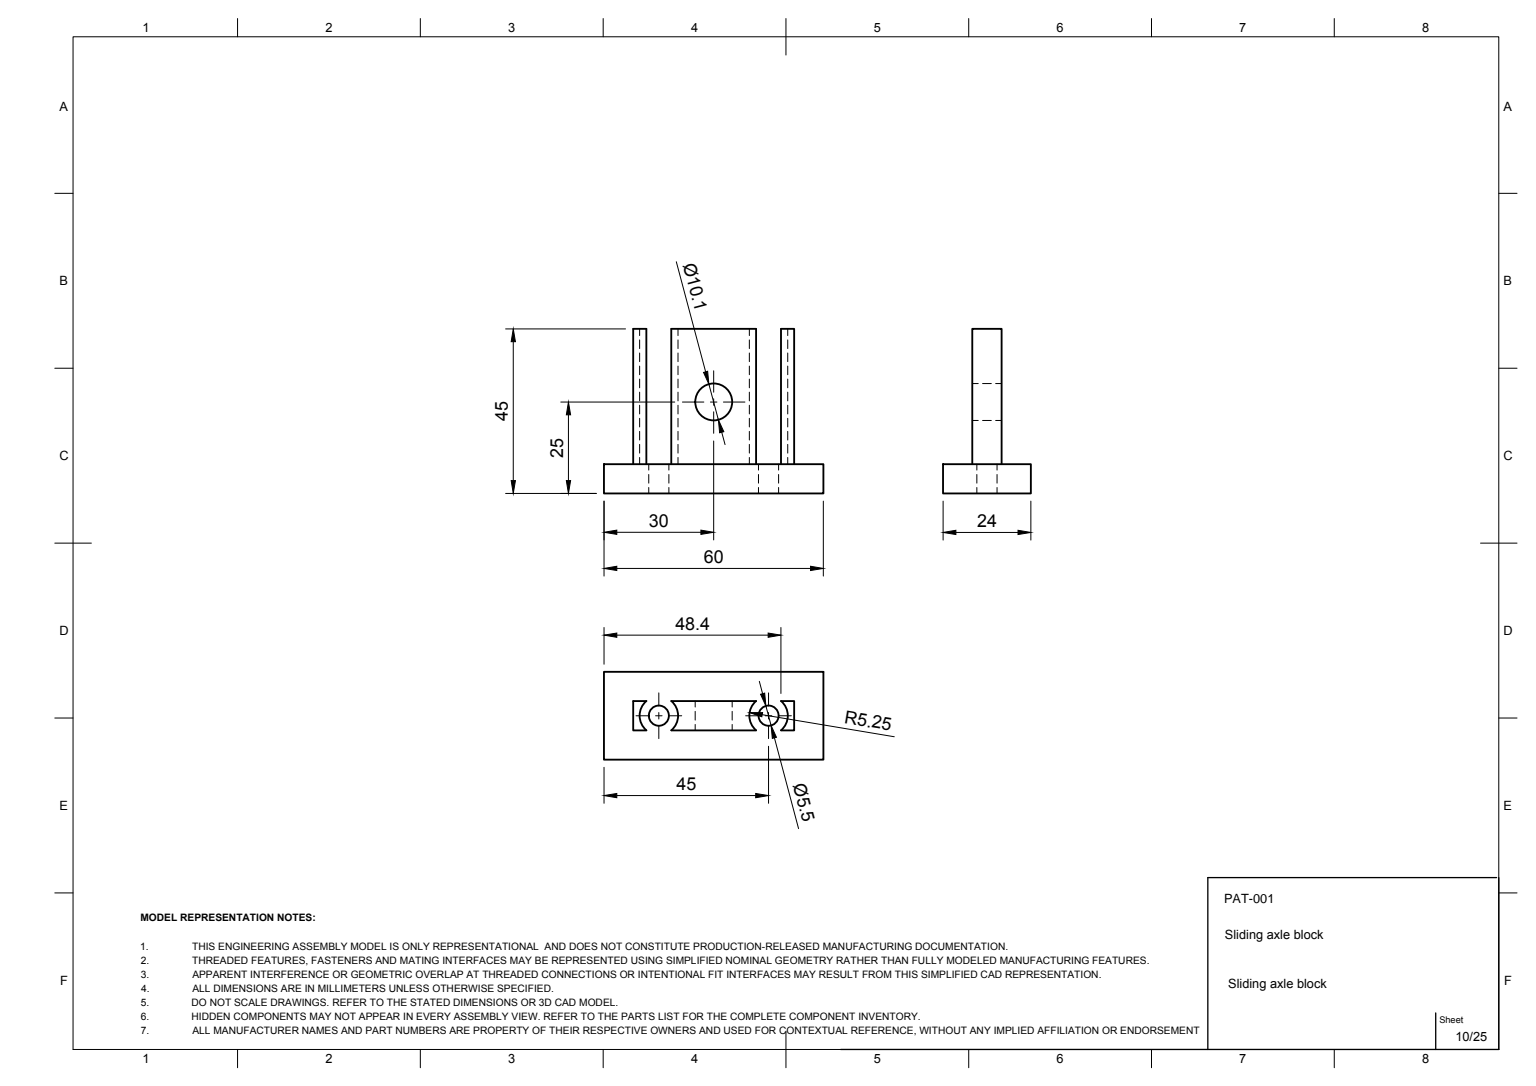
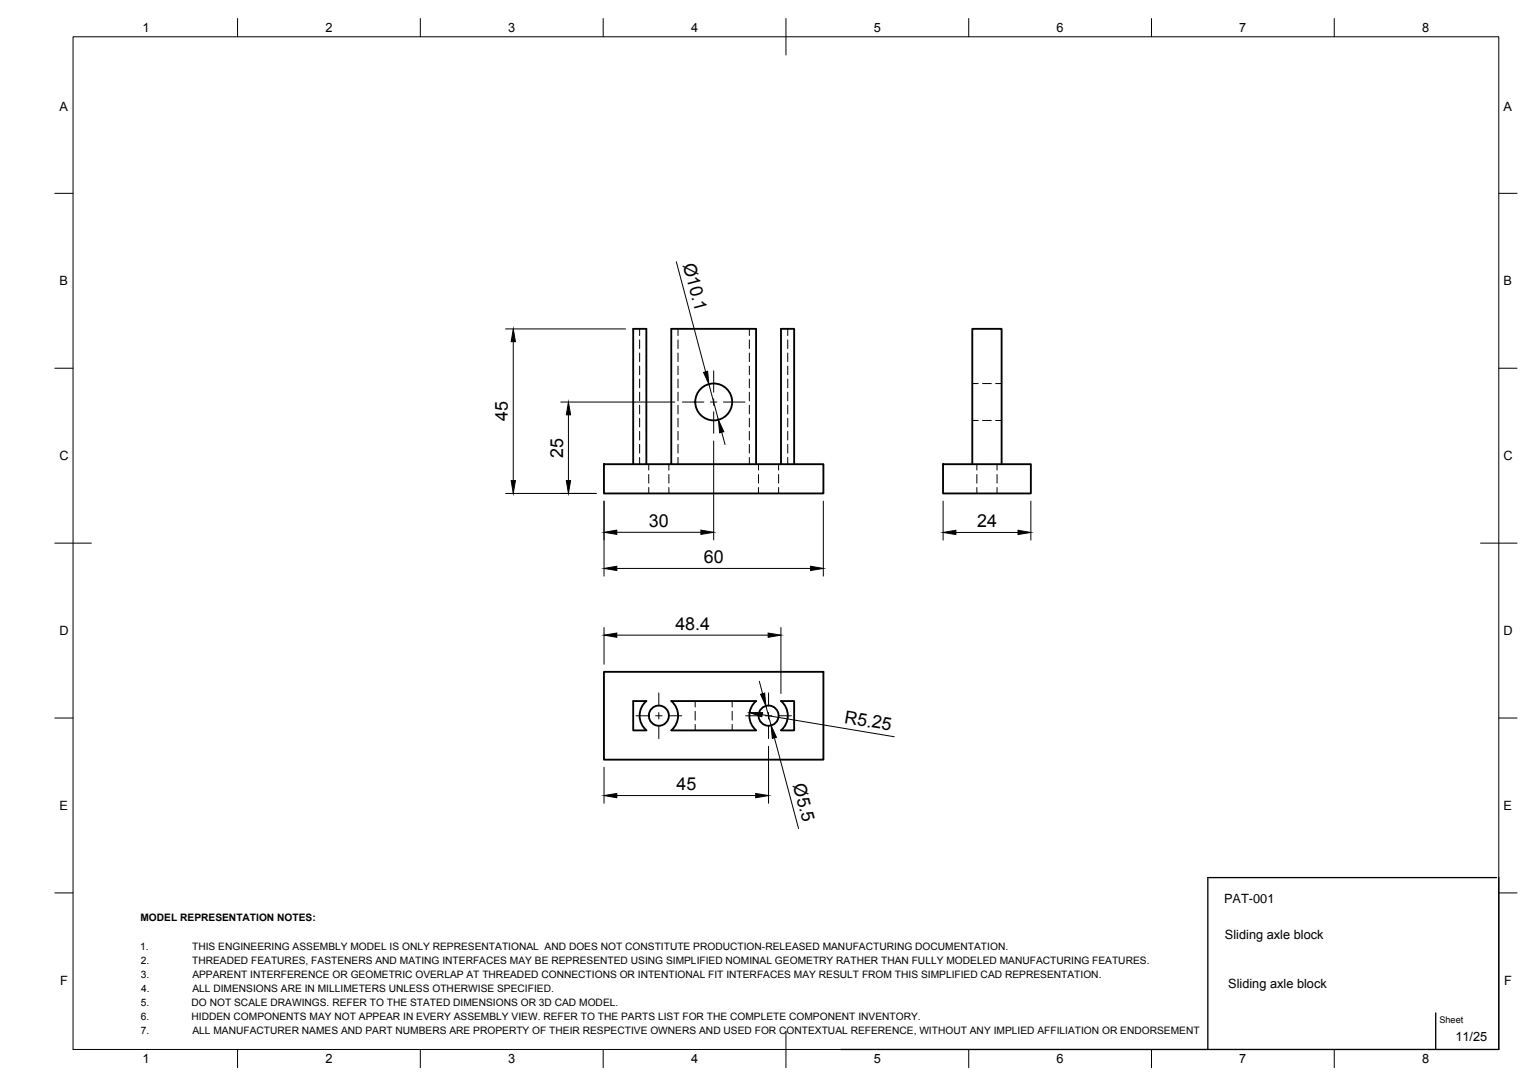
ISO-10303-21;
HEADER;
/* Generated by software containing ST-Developer
 * from STEP Tools, Inc. (www.steptools.com) 
 */

FILE_DESCRIPTION(
/* description */ ('PAT-001'),
/* implementation_level */ '2;1');

FILE_NAME(
/* name */ 'Sliding axle block.step',
/* time_stamp */ '2026-10-29T17:07:15-07:00',
/* author */ (''),
/* organization */ (''),
/* preprocessor_version */ 'ST-DEVELOPER v20.2',
/* originating_system */ 'Autodesk Translation Framework v15.17.0.0',
/* authorisation */ '');

FILE_SCHEMA (('AUTOMOTIVE_DESIGN { 1 0 10303 214 3 1 1 }'));
ENDSEC;

DATA;
#10=MECHANICAL_DESIGN_GEOMETRIC_PRESENTATION_REPRESENTATION('',(#391),#9622);
#333=SHAPE_REPRESENTATION_RELATIONSHIP('SRR','None',#9757,#358);
#358=ADVANCED_BREP_SHAPE_REPRESENTATION('',(#424),#9606);
#391=STYLED_ITEM('',(#9962),#424);
#424=MANIFOLD_SOLID_BREP('Body1',#5216);
#458=FACE_BOUND('',#1114,.T.);
#459=FACE_BOUND('',#1119,.T.);
#460=FACE_BOUND('',#1135,.T.);
#461=FACE_BOUND('',#1136,.T.);
#462=FACE_BOUND('',#1137,.T.);
#463=FACE_BOUND('',#1138,.T.);
#464=FACE_BOUND('',#1139,.T.);
#465=FACE_BOUND('',#1141,.T.);
#466=FACE_BOUND('',#1142,.T.);
#559=PLANE('',#5710);
#560=PLANE('',#5711);
#561=PLANE('',#5713);
#562=PLANE('',#5714);
#563=PLANE('',#5716);
#564=PLANE('',#5717);
#565=PLANE('',#5727);
#566=PLANE('',#5728);
#567=PLANE('',#5729);
#568=PLANE('',#5734);
#569=PLANE('',#5735);
#570=PLANE('',#5736);
#571=PLANE('',#5737);
#572=PLANE('',#5738);
#573=PLANE('',#5739);
#574=PLANE('',#5740);
#575=PLANE('',#5741);
#793=FACE_OUTER_BOUND('',#1110,.T.);
#794=FACE_OUTER_BOUND('',#1111,.T.);
#795=FACE_OUTER_BOUND('',#1112,.T.);
#796=FACE_OUTER_BOUND('',#1113,.T.);
#797=FACE_OUTER_BOUND('',#1115,.T.);
#798=FACE_OUTER_BOUND('',#1116,.T.);
#799=FACE_OUTER_BOUND('',#1117,.T.);
#800=FACE_OUTER_BOUND('',#1118,.T.);
#801=FACE_OUTER_BOUND('',#1120,.T.);
#802=FACE_OUTER_BOUND('',#1121,.T.);
#803=FACE_OUTER_BOUND('',#1122,.T.);
#804=FACE_OUTER_BOUND('',#1123,.T.);
#805=FACE_OUTER_BOUND('',#1124,.T.);
#806=FACE_OUTER_BOUND('',#1125,.T.);
#807=FACE_OUTER_BOUND('',#1126,.T.);
#808=FACE_OUTER_BOUND('',#1127,.T.);
#809=FACE_OUTER_BOUND('',#1128,.T.);
#810=FACE_OUTER_BOUND('',#1129,.T.);
#811=FACE_OUTER_BOUND('',#1130,.T.);
#812=FACE_OUTER_BOUND('',#1131,.T.);
#813=FACE_OUTER_BOUND('',#1132,.T.);
#814=FACE_OUTER_BOUND('',#1133,.T.);
#815=FACE_OUTER_BOUND('',#1134,.T.);
#816=FACE_OUTER_BOUND('',#1140,.T.);
#1110=EDGE_LOOP('',(#3807,#3808,#3809,#3810));
#1111=EDGE_LOOP('',(#3811,#3812,#3813,#3814));
#1112=EDGE_LOOP('',(#3815,#3816,#3817,#3818));
#1113=EDGE_LOOP('',(#3819,#3820,#3821,#3822));
#1114=EDGE_LOOP('',(#3823));
#1115=EDGE_LOOP('',(#3824,#3825,#3826,#3827));
#1116=EDGE_LOOP('',(#3828,#3829,#3830,#3831));
#1117=EDGE_LOOP('',(#3832,#3833,#3834,#3835));
#1118=EDGE_LOOP('',(#3836,#3837,#3838,#3839));
#1119=EDGE_LOOP('',(#3840));
#1120=EDGE_LOOP('',(#3841,#3842,#3843,#3844));
#1121=EDGE_LOOP('',(#3845,#3846,#3847,#3848));
#1122=EDGE_LOOP('',(#3849,#3850,#3851,#3852));
#1123=EDGE_LOOP('',(#3853,#3854,#3855,#3856));
#1124=EDGE_LOOP('',(#3857,#3858,#3859,#3860));
#1125=EDGE_LOOP('',(#3861,#3862,#3863,#3864));
#1126=EDGE_LOOP('',(#3865,#3866,#3867,#3868));
#1127=EDGE_LOOP('',(#3869,#3870,#3871,#3872));
#1128=EDGE_LOOP('',(#3873,#3874,#3875,#3876));
#1129=EDGE_LOOP('',(#3877,#3878,#3879,#3880));
#1130=EDGE_LOOP('',(#3881,#3882,#3883,#3884));
#1131=EDGE_LOOP('',(#3885,#3886,#3887,#3888));
#1132=EDGE_LOOP('',(#3889,#3890,#3891,#3892));
#1133=EDGE_LOOP('',(#3893,#3894,#3895,#3896));
#1134=EDGE_LOOP('',(#3897,#3898,#3899,#3900));
#1135=EDGE_LOOP('',(#3901,#3902,#3903,#3904));
#1136=EDGE_LOOP('',(#3905));
#1137=EDGE_LOOP('',(#3906,#3907,#3908,#3909));
#1138=EDGE_LOOP('',(#3910));
#1139=EDGE_LOOP('',(#3911,#3912,#3913,#3914));
#1140=EDGE_LOOP('',(#3915,#3916,#3917,#3918));
#1141=EDGE_LOOP('',(#3919));
#1142=EDGE_LOOP('',(#3920));
#1427=LINE('',#8397,#1832);
#1428=LINE('',#8401,#1833);
#1429=LINE('',#8406,#1834);
#1430=LINE('',#8410,#1835);
#1431=LINE('',#8414,#1836);
#1432=LINE('',#8416,#1837);
#1433=LINE('',#8417,#1838);
#1434=LINE('',#8420,#1839);
#1435=LINE('',#8422,#1840);
#1436=LINE('',#8423,#1841);
#1437=LINE('',#8428,#1842);
#1438=LINE('',#8429,#1843);
#1439=LINE('',#8432,#1844);
#1440=LINE('',#8436,#1845);
#1441=LINE('',#8437,#1846);
#1442=LINE('',#8440,#1847);
#1443=LINE('',#8441,#1848);
#1444=LINE('',#8448,#1849);
#1445=LINE('',#8453,#1850);
#1446=LINE('',#8457,#1851);
#1447=LINE('',#8463,#1852);
#1448=LINE('',#8465,#1853);
#1449=LINE('',#8466,#1854);
#1450=LINE('',#8469,#1855);
#1451=LINE('',#8470,#1856);
#1452=LINE('',#8473,#1857);
#1453=LINE('',#8474,#1858);
#1454=LINE('',#8479,#1859);
#1455=LINE('',#8482,#1860);
#1456=LINE('',#8484,#1861);
#1457=LINE('',#8486,#1862);
#1458=LINE('',#8490,#1863);
#1459=LINE('',#8492,#1864);
#1460=LINE('',#8494,#1865);
#1461=LINE('',#8495,#1866);
#1462=LINE('',#8498,#1867);
#1463=LINE('',#8500,#1868);
#1464=LINE('',#8501,#1869);
#1465=LINE('',#8504,#1870);
#1466=LINE('',#8506,#1871);
#1467=LINE('',#8507,#1872);
#1468=LINE('',#8509,#1873);
#1469=LINE('',#8510,#1874);
#1832=VECTOR('',#6528,1.);
#1833=VECTOR('',#6531,1.);
#1834=VECTOR('',#6536,1.);
#1835=VECTOR('',#6539,1.);
#1836=VECTOR('',#6544,1.);
#1837=VECTOR('',#6545,1.);
#1838=VECTOR('',#6546,1.);
#1839=VECTOR('',#6549,1.);
#1840=VECTOR('',#6550,1.);
#1841=VECTOR('',#6551,1.);
#1842=VECTOR('',#6556,1.);
#1843=VECTOR('',#6557,1.);
#1844=VECTOR('',#6560,1.);
#1845=VECTOR('',#6565,1.);
#1846=VECTOR('',#6566,1.);
#1847=VECTOR('',#6569,1.);
#1848=VECTOR('',#6570,1.);
#1849=VECTOR('',#6577,0.275);
#1850=VECTOR('',#6582,1.);
#1851=VECTOR('',#6585,1.);
#1852=VECTOR('',#6594,1.);
#1853=VECTOR('',#6595,1.);
#1854=VECTOR('',#6596,1.);
#1855=VECTOR('',#6599,1.);
#1856=VECTOR('',#6600,1.);
#1857=VECTOR('',#6603,1.);
#1858=VECTOR('',#6604,1.);
#1859=VECTOR('',#6609,0.275);
#1860=VECTOR('',#6614,0.505);
#1861=VECTOR('',#6617,1.);
#1862=VECTOR('',#6620,1.);
#1863=VECTOR('',#6623,1.);
#1864=VECTOR('',#6624,1.);
#1865=VECTOR('',#6625,1.);
#1866=VECTOR('',#6626,1.);
#1867=VECTOR('',#6629,1.);
#1868=VECTOR('',#6630,1.);
#1869=VECTOR('',#6631,1.);
#1870=VECTOR('',#6634,1.);
#1871=VECTOR('',#6635,1.);
#1872=VECTOR('',#6636,1.);
#1873=VECTOR('',#6639,1.);
#1874=VECTOR('',#6640,1.);
#2306=CIRCLE('',#5705,0.525);
#2307=CIRCLE('',#5706,0.525);
#2308=CIRCLE('',#5708,0.525);
#2309=CIRCLE('',#5709,0.525);
#2310=CIRCLE('',#5712,0.505);
#2311=CIRCLE('',#5715,0.525);
#2312=CIRCLE('',#5718,0.505);
#2313=CIRCLE('',#5720,0.275);
#2314=CIRCLE('',#5721,0.275);
#2315=CIRCLE('',#5723,0.525);
#2316=CIRCLE('',#5724,0.525);
#2317=CIRCLE('',#5726,0.525);
#2318=CIRCLE('',#5731,0.275);
#2319=CIRCLE('',#5732,0.275);
#2526=VERTEX_POINT('',#8395);
#2527=VERTEX_POINT('',#8396);
#2528=VERTEX_POINT('',#8398);
#2529=VERTEX_POINT('',#8400);
#2530=VERTEX_POINT('',#8404);
#2531=VERTEX_POINT('',#8405);
#2532=VERTEX_POINT('',#8407);
#2533=VERTEX_POINT('',#8409);
#2534=VERTEX_POINT('',#8413);
#2535=VERTEX_POINT('',#8415);
#2536=VERTEX_POINT('',#8419);
#2537=VERTEX_POINT('',#8421);
#2538=VERTEX_POINT('',#8424);
#2539=VERTEX_POINT('',#8427);
#2540=VERTEX_POINT('',#8431);
#2541=VERTEX_POINT('',#8435);
#2542=VERTEX_POINT('',#8439);
#2543=VERTEX_POINT('',#8442);
#2544=VERTEX_POINT('',#8445);
#2545=VERTEX_POINT('',#8447);
#2546=VERTEX_POINT('',#8451);
#2547=VERTEX_POINT('',#8452);
#2548=VERTEX_POINT('',#8454);
#2549=VERTEX_POINT('',#8456);
#2550=VERTEX_POINT('',#8462);
#2551=VERTEX_POINT('',#8464);
#2552=VERTEX_POINT('',#8468);
#2553=VERTEX_POINT('',#8472);
#2554=VERTEX_POINT('',#8476);
#2555=VERTEX_POINT('',#8478);
#2556=VERTEX_POINT('',#8488);
#2557=VERTEX_POINT('',#8489);
#2558=VERTEX_POINT('',#8491);
#2559=VERTEX_POINT('',#8493);
#2560=VERTEX_POINT('',#8497);
#2561=VERTEX_POINT('',#8499);
#2562=VERTEX_POINT('',#8503);
#2563=VERTEX_POINT('',#8505);
#3007=EDGE_CURVE('',#2526,#2527,#1427,.T.);
#3008=EDGE_CURVE('',#2528,#2526,#2306,.T.);
#3009=EDGE_CURVE('',#2529,#2528,#1428,.T.);
#3010=EDGE_CURVE('',#2527,#2529,#2307,.T.);
#3011=EDGE_CURVE('',#2530,#2531,#1429,.T.);
#3012=EDGE_CURVE('',#2532,#2530,#2308,.T.);
#3013=EDGE_CURVE('',#2533,#2532,#1430,.T.);
#3014=EDGE_CURVE('',#2531,#2533,#2309,.T.);
#3015=EDGE_CURVE('',#2534,#2527,#1431,.T.);
#3016=EDGE_CURVE('',#2534,#2535,#1432,.T.);
#3017=EDGE_CURVE('',#2535,#2526,#1433,.T.);
#3018=EDGE_CURVE('',#2531,#2536,#1434,.T.);
#3019=EDGE_CURVE('',#2536,#2537,#1435,.T.);
#3020=EDGE_CURVE('',#2530,#2537,#1436,.T.);
#3021=EDGE_CURVE('',#2538,#2538,#2310,.T.);
#3022=EDGE_CURVE('',#2535,#2539,#1437,.T.);
#3023=EDGE_CURVE('',#2528,#2539,#1438,.T.);
#3024=EDGE_CURVE('',#2540,#2533,#1439,.T.);
#3025=EDGE_CURVE('',#2540,#2536,#2311,.T.);
#3026=EDGE_CURVE('',#2539,#2541,#1440,.T.);
#3027=EDGE_CURVE('',#2529,#2541,#1441,.T.);
#3028=EDGE_CURVE('',#2542,#2532,#1442,.T.);
#3029=EDGE_CURVE('',#2542,#2540,#1443,.T.);
#3030=EDGE_CURVE('',#2543,#2543,#2312,.T.);
#3031=EDGE_CURVE('',#2544,#2544,#2313,.T.);
#3032=EDGE_CURVE('',#2544,#2545,#1444,.T.);
#3033=EDGE_CURVE('',#2545,#2545,#2314,.T.);
#3034=EDGE_CURVE('',#2546,#2547,#1445,.T.);
#3035=EDGE_CURVE('',#2548,#2546,#2315,.T.);
#3036=EDGE_CURVE('',#2549,#2548,#1446,.T.);
#3037=EDGE_CURVE('',#2547,#2549,#2316,.T.);
#3038=EDGE_CURVE('',#2537,#2542,#2317,.T.);
#3039=EDGE_CURVE('',#2550,#2547,#1447,.T.);
#3040=EDGE_CURVE('',#2550,#2551,#1448,.T.);
#3041=EDGE_CURVE('',#2551,#2546,#1449,.T.);
#3042=EDGE_CURVE('',#2552,#2551,#1450,.T.);
#3043=EDGE_CURVE('',#2548,#2552,#1451,.T.);
#3044=EDGE_CURVE('',#2552,#2553,#1452,.T.);
#3045=EDGE_CURVE('',#2549,#2553,#1453,.T.);
#3046=EDGE_CURVE('',#2554,#2554,#2318,.T.);
#3047=EDGE_CURVE('',#2554,#2555,#1454,.T.);
#3048=EDGE_CURVE('',#2555,#2555,#2319,.T.);
#3049=EDGE_CURVE('',#2538,#2543,#1455,.T.);
#3050=EDGE_CURVE('',#2541,#2534,#1456,.T.);
#3051=EDGE_CURVE('',#2553,#2550,#1457,.T.);
#3052=EDGE_CURVE('',#2556,#2557,#1458,.T.);
#3053=EDGE_CURVE('',#2557,#2558,#1459,.T.);
#3054=EDGE_CURVE('',#2559,#2558,#1460,.T.);
#3055=EDGE_CURVE('',#2556,#2559,#1461,.T.);
#3056=EDGE_CURVE('',#2560,#2556,#1462,.T.);
#3057=EDGE_CURVE('',#2561,#2559,#1463,.T.);
#3058=EDGE_CURVE('',#2560,#2561,#1464,.T.);
#3059=EDGE_CURVE('',#2562,#2560,#1465,.T.);
#3060=EDGE_CURVE('',#2563,#2561,#1466,.T.);
#3061=EDGE_CURVE('',#2562,#2563,#1467,.T.);
#3062=EDGE_CURVE('',#2557,#2562,#1468,.T.);
#3063=EDGE_CURVE('',#2558,#2563,#1469,.T.);
#3807=ORIENTED_EDGE('',*,*,#3007,.F.);
#3808=ORIENTED_EDGE('',*,*,#3008,.F.);
#3809=ORIENTED_EDGE('',*,*,#3009,.F.);
#3810=ORIENTED_EDGE('',*,*,#3010,.F.);
#3811=ORIENTED_EDGE('',*,*,#3011,.F.);
#3812=ORIENTED_EDGE('',*,*,#3012,.F.);
#3813=ORIENTED_EDGE('',*,*,#3013,.F.);
#3814=ORIENTED_EDGE('',*,*,#3014,.F.);
#3815=ORIENTED_EDGE('',*,*,#3007,.T.);
#3816=ORIENTED_EDGE('',*,*,#3015,.F.);
#3817=ORIENTED_EDGE('',*,*,#3016,.T.);
#3818=ORIENTED_EDGE('',*,*,#3017,.T.);
#3819=ORIENTED_EDGE('',*,*,#3011,.T.);
#3820=ORIENTED_EDGE('',*,*,#3018,.T.);
#3821=ORIENTED_EDGE('',*,*,#3019,.T.);
#3822=ORIENTED_EDGE('',*,*,#3020,.F.);
#3823=ORIENTED_EDGE('',*,*,#3021,.T.);
#3824=ORIENTED_EDGE('',*,*,#3008,.T.);
#3825=ORIENTED_EDGE('',*,*,#3017,.F.);
#3826=ORIENTED_EDGE('',*,*,#3022,.T.);
#3827=ORIENTED_EDGE('',*,*,#3023,.F.);
#3828=ORIENTED_EDGE('',*,*,#3014,.T.);
#3829=ORIENTED_EDGE('',*,*,#3024,.F.);
#3830=ORIENTED_EDGE('',*,*,#3025,.T.);
#3831=ORIENTED_EDGE('',*,*,#3018,.F.);
#3832=ORIENTED_EDGE('',*,*,#3009,.T.);
#3833=ORIENTED_EDGE('',*,*,#3023,.T.);
#3834=ORIENTED_EDGE('',*,*,#3026,.T.);
#3835=ORIENTED_EDGE('',*,*,#3027,.F.);
#3836=ORIENTED_EDGE('',*,*,#3013,.T.);
#3837=ORIENTED_EDGE('',*,*,#3028,.F.);
#3838=ORIENTED_EDGE('',*,*,#3029,.T.);
#3839=ORIENTED_EDGE('',*,*,#3024,.T.);
#3840=ORIENTED_EDGE('',*,*,#3030,.T.);
#3841=ORIENTED_EDGE('',*,*,#3031,.F.);
#3842=ORIENTED_EDGE('',*,*,#3032,.T.);
#3843=ORIENTED_EDGE('',*,*,#3033,.T.);
#3844=ORIENTED_EDGE('',*,*,#3032,.F.);
#3845=ORIENTED_EDGE('',*,*,#3034,.F.);
#3846=ORIENTED_EDGE('',*,*,#3035,.F.);
#3847=ORIENTED_EDGE('',*,*,#3036,.F.);
#3848=ORIENTED_EDGE('',*,*,#3037,.F.);
#3849=ORIENTED_EDGE('',*,*,#3029,.F.);
#3850=ORIENTED_EDGE('',*,*,#3038,.F.);
#3851=ORIENTED_EDGE('',*,*,#3019,.F.);
#3852=ORIENTED_EDGE('',*,*,#3025,.F.);
#3853=ORIENTED_EDGE('',*,*,#3034,.T.);
#3854=ORIENTED_EDGE('',*,*,#3039,.F.);
#3855=ORIENTED_EDGE('',*,*,#3040,.T.);
#3856=ORIENTED_EDGE('',*,*,#3041,.T.);
#3857=ORIENTED_EDGE('',*,*,#3035,.T.);
#3858=ORIENTED_EDGE('',*,*,#3041,.F.);
#3859=ORIENTED_EDGE('',*,*,#3042,.F.);
#3860=ORIENTED_EDGE('',*,*,#3043,.F.);
#3861=ORIENTED_EDGE('',*,*,#3036,.T.);
#3862=ORIENTED_EDGE('',*,*,#3043,.T.);
#3863=ORIENTED_EDGE('',*,*,#3044,.T.);
#3864=ORIENTED_EDGE('',*,*,#3045,.F.);
#3865=ORIENTED_EDGE('',*,*,#3046,.F.);
#3866=ORIENTED_EDGE('',*,*,#3047,.T.);
#3867=ORIENTED_EDGE('',*,*,#3048,.T.);
#3868=ORIENTED_EDGE('',*,*,#3047,.F.);
#3869=ORIENTED_EDGE('',*,*,#3021,.F.);
#3870=ORIENTED_EDGE('',*,*,#3049,.T.);
#3871=ORIENTED_EDGE('',*,*,#3030,.F.);
#3872=ORIENTED_EDGE('',*,*,#3049,.F.);
#3873=ORIENTED_EDGE('',*,*,#3050,.F.);
#3874=ORIENTED_EDGE('',*,*,#3026,.F.);
#3875=ORIENTED_EDGE('',*,*,#3022,.F.);
#3876=ORIENTED_EDGE('',*,*,#3016,.F.);
#3877=ORIENTED_EDGE('',*,*,#3051,.F.);
#3878=ORIENTED_EDGE('',*,*,#3044,.F.);
#3879=ORIENTED_EDGE('',*,*,#3042,.T.);
#3880=ORIENTED_EDGE('',*,*,#3040,.F.);
#3881=ORIENTED_EDGE('',*,*,#3052,.T.);
#3882=ORIENTED_EDGE('',*,*,#3053,.T.);
#3883=ORIENTED_EDGE('',*,*,#3054,.F.);
#3884=ORIENTED_EDGE('',*,*,#3055,.F.);
#3885=ORIENTED_EDGE('',*,*,#3056,.T.);
#3886=ORIENTED_EDGE('',*,*,#3055,.T.);
#3887=ORIENTED_EDGE('',*,*,#3057,.F.);
#3888=ORIENTED_EDGE('',*,*,#3058,.F.);
#3889=ORIENTED_EDGE('',*,*,#3059,.T.);
#3890=ORIENTED_EDGE('',*,*,#3058,.T.);
#3891=ORIENTED_EDGE('',*,*,#3060,.F.);
#3892=ORIENTED_EDGE('',*,*,#3061,.F.);
#3893=ORIENTED_EDGE('',*,*,#3062,.T.);
#3894=ORIENTED_EDGE('',*,*,#3061,.T.);
#3895=ORIENTED_EDGE('',*,*,#3063,.F.);
#3896=ORIENTED_EDGE('',*,*,#3053,.F.);
#3897=ORIENTED_EDGE('',*,*,#3063,.T.);
#3898=ORIENTED_EDGE('',*,*,#3060,.T.);
#3899=ORIENTED_EDGE('',*,*,#3057,.T.);
#3900=ORIENTED_EDGE('',*,*,#3054,.T.);
#3901=ORIENTED_EDGE('',*,*,#3020,.T.);
#3902=ORIENTED_EDGE('',*,*,#3038,.T.);
#3903=ORIENTED_EDGE('',*,*,#3028,.T.);
#3904=ORIENTED_EDGE('',*,*,#3012,.T.);
#3905=ORIENTED_EDGE('',*,*,#3033,.F.);
#3906=ORIENTED_EDGE('',*,*,#3010,.T.);
#3907=ORIENTED_EDGE('',*,*,#3027,.T.);
#3908=ORIENTED_EDGE('',*,*,#3050,.T.);
#3909=ORIENTED_EDGE('',*,*,#3015,.T.);
#3910=ORIENTED_EDGE('',*,*,#3048,.F.);
#3911=ORIENTED_EDGE('',*,*,#3037,.T.);
#3912=ORIENTED_EDGE('',*,*,#3045,.T.);
#3913=ORIENTED_EDGE('',*,*,#3051,.T.);
#3914=ORIENTED_EDGE('',*,*,#3039,.T.);
#3915=ORIENTED_EDGE('',*,*,#3062,.F.);
#3916=ORIENTED_EDGE('',*,*,#3052,.F.);
#3917=ORIENTED_EDGE('',*,*,#3056,.F.);
#3918=ORIENTED_EDGE('',*,*,#3059,.F.);
#3919=ORIENTED_EDGE('',*,*,#3031,.T.);
#3920=ORIENTED_EDGE('',*,*,#3046,.T.);
#4852=CYLINDRICAL_SURFACE('',#5704,0.525);
#4853=CYLINDRICAL_SURFACE('',#5707,0.525);
#4854=CYLINDRICAL_SURFACE('',#5719,0.275);
#4855=CYLINDRICAL_SURFACE('',#5722,0.525);
#4856=CYLINDRICAL_SURFACE('',#5725,0.525);
#4857=CYLINDRICAL_SURFACE('',#5730,0.275);
#4858=CYLINDRICAL_SURFACE('',#5733,0.505);
#4980=ADVANCED_FACE('',(#793),#4852,.F.);
#4981=ADVANCED_FACE('',(#794),#4853,.F.);
#4982=ADVANCED_FACE('',(#795),#559,.F.);
#4983=ADVANCED_FACE('',(#796,#458),#560,.F.);
#4984=ADVANCED_FACE('',(#797),#561,.T.);
#4985=ADVANCED_FACE('',(#798),#562,.T.);
#4986=ADVANCED_FACE('',(#799),#563,.T.);
#4987=ADVANCED_FACE('',(#800,#459),#564,.T.);
#4988=ADVANCED_FACE('',(#801),#4854,.F.);
#4989=ADVANCED_FACE('',(#802),#4855,.F.);
#4990=ADVANCED_FACE('',(#803),#4856,.F.);
#4991=ADVANCED_FACE('',(#804),#565,.T.);
#4992=ADVANCED_FACE('',(#805),#566,.T.);
#4993=ADVANCED_FACE('',(#806),#567,.F.);
#4994=ADVANCED_FACE('',(#807),#4857,.F.);
#4995=ADVANCED_FACE('',(#808),#4858,.F.);
#4996=ADVANCED_FACE('',(#809),#568,.T.);
#4997=ADVANCED_FACE('',(#810),#569,.T.);
#4998=ADVANCED_FACE('',(#811),#570,.T.);
#4999=ADVANCED_FACE('',(#812),#571,.T.);
#5000=ADVANCED_FACE('',(#813),#572,.T.);
#5001=ADVANCED_FACE('',(#814),#573,.T.);
#5002=ADVANCED_FACE('',(#815,#460,#461,#462,#463,#464),#574,.T.);
#5003=ADVANCED_FACE('',(#816,#465,#466),#575,.F.);
#5216=CLOSED_SHELL('',(#4980,#4981,#4982,#4983,#4984,#4985,#4986,#4987,
#4988,#4989,#4990,#4991,#4992,#4993,#4994,#4995,#4996,#4997,#4998,#4999,
#5000,#5001,#5002,#5003));
#5703=AXIS2_PLACEMENT_3D('',#8393,#6524,#6525);
#5704=AXIS2_PLACEMENT_3D('',#8394,#6526,#6527);
#5705=AXIS2_PLACEMENT_3D('',#8399,#6529,#6530);
#5706=AXIS2_PLACEMENT_3D('',#8402,#6532,#6533);
#5707=AXIS2_PLACEMENT_3D('',#8403,#6534,#6535);
#5708=AXIS2_PLACEMENT_3D('',#8408,#6537,#6538);
#5709=AXIS2_PLACEMENT_3D('',#8411,#6540,#6541);
#5710=AXIS2_PLACEMENT_3D('',#8412,#6542,#6543);
#5711=AXIS2_PLACEMENT_3D('',#8418,#6547,#6548);
#5712=AXIS2_PLACEMENT_3D('',#8425,#6552,#6553);
#5713=AXIS2_PLACEMENT_3D('',#8426,#6554,#6555);
#5714=AXIS2_PLACEMENT_3D('',#8430,#6558,#6559);
#5715=AXIS2_PLACEMENT_3D('',#8433,#6561,#6562);
#5716=AXIS2_PLACEMENT_3D('',#8434,#6563,#6564);
#5717=AXIS2_PLACEMENT_3D('',#8438,#6567,#6568);
#5718=AXIS2_PLACEMENT_3D('',#8443,#6571,#6572);
#5719=AXIS2_PLACEMENT_3D('',#8444,#6573,#6574);
#5720=AXIS2_PLACEMENT_3D('',#8446,#6575,#6576);
#5721=AXIS2_PLACEMENT_3D('',#8449,#6578,#6579);
#5722=AXIS2_PLACEMENT_3D('',#8450,#6580,#6581);
#5723=AXIS2_PLACEMENT_3D('',#8455,#6583,#6584);
#5724=AXIS2_PLACEMENT_3D('',#8458,#6586,#6587);
#5725=AXIS2_PLACEMENT_3D('',#8459,#6588,#6589);
#5726=AXIS2_PLACEMENT_3D('',#8460,#6590,#6591);
#5727=AXIS2_PLACEMENT_3D('',#8461,#6592,#6593);
#5728=AXIS2_PLACEMENT_3D('',#8467,#6597,#6598);
#5729=AXIS2_PLACEMENT_3D('',#8471,#6601,#6602);
#5730=AXIS2_PLACEMENT_3D('',#8475,#6605,#6606);
#5731=AXIS2_PLACEMENT_3D('',#8477,#6607,#6608);
#5732=AXIS2_PLACEMENT_3D('',#8480,#6610,#6611);
#5733=AXIS2_PLACEMENT_3D('',#8481,#6612,#6613);
#5734=AXIS2_PLACEMENT_3D('',#8483,#6615,#6616);
#5735=AXIS2_PLACEMENT_3D('',#8485,#6618,#6619);
#5736=AXIS2_PLACEMENT_3D('',#8487,#6621,#6622);
#5737=AXIS2_PLACEMENT_3D('',#8496,#6627,#6628);
#5738=AXIS2_PLACEMENT_3D('',#8502,#6632,#6633);
#5739=AXIS2_PLACEMENT_3D('',#8508,#6637,#6638);
#5740=AXIS2_PLACEMENT_3D('',#8511,#6641,#6642);
#5741=AXIS2_PLACEMENT_3D('',#8512,#6643,#6644);
#6524=DIRECTION('axis',(0.,0.,1.));
#6525=DIRECTION('refdir',(1.,0.,0.));
#6526=DIRECTION('center_axis',(0.,0.,1.));
#6527=DIRECTION('ref_axis',(1.,0.,0.));
#6528=DIRECTION('',(0.,0.,-1.));
#6529=DIRECTION('center_axis',(0.,0.,-1.));
#6530=DIRECTION('ref_axis',(1.,0.,0.));
#6531=DIRECTION('',(0.,0.,1.));
#6532=DIRECTION('center_axis',(0.,0.,1.));
#6533=DIRECTION('ref_axis',(1.,0.,0.));
#6534=DIRECTION('center_axis',(0.,0.,1.));
#6535=DIRECTION('ref_axis',(-1.,-1.01064309961486E-15,0.));
#6536=DIRECTION('',(0.,0.,1.));
#6537=DIRECTION('center_axis',(0.,0.,1.));
#6538=DIRECTION('ref_axis',(1.,0.,0.));
#6539=DIRECTION('',(0.,0.,-1.));
#6540=DIRECTION('center_axis',(0.,0.,-1.));
#6541=DIRECTION('ref_axis',(1.,0.,0.));
#6542=DIRECTION('center_axis',(0.,1.,0.));
#6543=DIRECTION('ref_axis',(1.,0.,0.));
#6544=DIRECTION('',(-1.,0.,0.));
#6545=DIRECTION('',(0.,0.,1.));
#6546=DIRECTION('',(-1.,0.,0.));
#6547=DIRECTION('center_axis',(0.,1.,0.));
#6548=DIRECTION('ref_axis',(1.,0.,0.));
#6549=DIRECTION('',(-1.,0.,0.));
#6550=DIRECTION('',(0.,0.,-1.));
#6551=DIRECTION('',(-1.,0.,0.));
#6552=DIRECTION('center_axis',(0.,1.,0.));
#6553=DIRECTION('ref_axis',(1.,0.,0.));
#6554=DIRECTION('center_axis',(0.,0.,1.));
#6555=DIRECTION('ref_axis',(1.,0.,0.));
#6556=DIRECTION('',(0.,1.,0.));
#6557=DIRECTION('',(1.,0.,0.));
#6558=DIRECTION('center_axis',(0.,0.,1.));
#6559=DIRECTION('ref_axis',(1.,0.,0.));
#6560=DIRECTION('',(1.,0.,0.));
#6561=DIRECTION('center_axis',(0.,0.,-1.));
#6562=DIRECTION('ref_axis',(1.,0.,0.));
#6563=DIRECTION('center_axis',(0.,1.,0.));
#6564=DIRECTION('ref_axis',(0.,0.,1.));
#6565=DIRECTION('',(0.,0.,-1.));
#6566=DIRECTION('',(1.,0.,0.));
#6567=DIRECTION('center_axis',(0.,1.,0.));
#6568=DIRECTION('ref_axis',(0.,0.,1.));
#6569=DIRECTION('',(1.,0.,0.));
#6570=DIRECTION('',(0.,0.,1.));
#6571=DIRECTION('center_axis',(0.,-1.,0.));
#6572=DIRECTION('ref_axis',(1.,0.,0.));
#6573=DIRECTION('center_axis',(0.,0.,1.));
#6574=DIRECTION('ref_axis',(1.,0.,0.));
#6575=DIRECTION('center_axis',(0.,0.,1.));
#6576=DIRECTION('ref_axis',(1.,0.,0.));
#6577=DIRECTION('',(0.,0.,1.));
#6578=DIRECTION('center_axis',(0.,0.,1.));
#6579=DIRECTION('ref_axis',(1.,0.,0.));
#6580=DIRECTION('center_axis',(0.,0.,1.));
#6581=DIRECTION('ref_axis',(-1.,-7.6571373978539E-16,0.));
#6582=DIRECTION('',(0.,0.,-1.));
#6583=DIRECTION('center_axis',(0.,0.,-1.));
#6584=DIRECTION('ref_axis',(1.,0.,0.));
#6585=DIRECTION('',(0.,0.,1.));
#6586=DIRECTION('center_axis',(0.,0.,1.));
#6587=DIRECTION('ref_axis',(1.,0.,0.));
#6588=DIRECTION('center_axis',(0.,0.,1.));
#6589=DIRECTION('ref_axis',(1.,0.,0.));
#6590=DIRECTION('center_axis',(0.,0.,1.));
#6591=DIRECTION('ref_axis',(1.,0.,0.));
#6592=DIRECTION('center_axis',(0.,1.,0.));
#6593=DIRECTION('ref_axis',(0.,0.,1.));
#6594=DIRECTION('',(1.,0.,0.));
#6595=DIRECTION('',(0.,0.,1.));
#6596=DIRECTION('',(1.,0.,0.));
#6597=DIRECTION('center_axis',(0.,0.,1.));
#6598=DIRECTION('ref_axis',(1.,0.,0.));
#6599=DIRECTION('',(0.,1.,0.));
#6600=DIRECTION('',(-1.,0.,0.));
#6601=DIRECTION('center_axis',(0.,1.,0.));
#6602=DIRECTION('ref_axis',(1.,0.,0.));
#6603=DIRECTION('',(0.,0.,-1.));
#6604=DIRECTION('',(-1.,0.,0.));
#6605=DIRECTION('center_axis',(0.,0.,1.));
#6606=DIRECTION('ref_axis',(1.,0.,0.));
#6607=DIRECTION('center_axis',(0.,0.,1.));
#6608=DIRECTION('ref_axis',(1.,0.,0.));
#6609=DIRECTION('',(0.,0.,1.));
#6610=DIRECTION('center_axis',(0.,0.,1.));
#6611=DIRECTION('ref_axis',(1.,0.,0.));
#6612=DIRECTION('center_axis',(0.,1.,0.));
#6613=DIRECTION('ref_axis',(1.,0.,0.));
#6614=DIRECTION('',(0.,1.,0.));
#6615=DIRECTION('center_axis',(1.,0.,0.));
#6616=DIRECTION('ref_axis',(0.,0.,-1.));
#6617=DIRECTION('',(0.,-1.,0.));
#6618=DIRECTION('center_axis',(-1.,0.,0.));
#6619=DIRECTION('ref_axis',(0.,0.,1.));
#6620=DIRECTION('',(0.,1.,0.));
#6621=DIRECTION('center_axis',(0.,1.,0.));
#6622=DIRECTION('ref_axis',(-1.,0.,0.));
#6623=DIRECTION('',(-1.,0.,0.));
#6624=DIRECTION('',(0.,0.,1.));
#6625=DIRECTION('',(-1.,0.,0.));
#6626=DIRECTION('',(0.,0.,1.));
#6627=DIRECTION('center_axis',(1.,0.,0.));
#6628=DIRECTION('ref_axis',(0.,1.,0.));
#6629=DIRECTION('',(0.,1.,0.));
#6630=DIRECTION('',(0.,1.,0.));
#6631=DIRECTION('',(0.,0.,1.));
#6632=DIRECTION('center_axis',(0.,-1.,0.));
#6633=DIRECTION('ref_axis',(1.,0.,0.));
#6634=DIRECTION('',(1.,0.,0.));
#6635=DIRECTION('',(1.,0.,0.));
#6636=DIRECTION('',(0.,0.,1.));
#6637=DIRECTION('center_axis',(-1.,0.,0.));
#6638=DIRECTION('ref_axis',(0.,-1.,0.));
#6639=DIRECTION('',(0.,-1.,0.));
#6640=DIRECTION('',(0.,-1.,0.));
#6641=DIRECTION('center_axis',(0.,0.,1.));
#6642=DIRECTION('ref_axis',(1.,0.,0.));
#6643=DIRECTION('center_axis',(0.,0.,1.));
#6644=DIRECTION('ref_axis',(1.,0.,0.));
#8393=CARTESIAN_POINT('',(0.,0.,0.));
#8394=CARTESIAN_POINT('Origin',(1.5,-2.,2.8));
#8395=CARTESIAN_POINT('',(1.84003676271839,-2.4,6.5));
#8396=CARTESIAN_POINT('',(1.84003676271839,-2.4,2.8));
#8397=CARTESIAN_POINT('',(1.84003676271839,-2.4,2.8));
#8398=CARTESIAN_POINT('',(1.84003676271839,-1.6,6.5));
#8399=CARTESIAN_POINT('Origin',(1.5,-2.,6.5));
#8400=CARTESIAN_POINT('',(1.84003676271839,-1.6,2.8));
#8401=CARTESIAN_POINT('',(1.84003676271839,-1.6,2.8));
#8402=CARTESIAN_POINT('Origin',(1.5,-2.,2.8));
#8403=CARTESIAN_POINT('Origin',(1.5,-2.,2.8));
#8404=CARTESIAN_POINT('',(1.15996323728161,-2.4,2.8));
#8405=CARTESIAN_POINT('',(1.15996323728161,-2.4,6.5));
#8406=CARTESIAN_POINT('',(1.15996323728161,-2.4,2.8));
#8407=CARTESIAN_POINT('',(1.15996323728161,-1.6,2.8));
#8408=CARTESIAN_POINT('Origin',(1.5,-2.,2.8));
#8409=CARTESIAN_POINT('',(1.15996323728161,-1.6,6.5));
#8410=CARTESIAN_POINT('',(1.15996323728161,-1.6,2.8));
#8411=CARTESIAN_POINT('Origin',(1.5,-2.,6.5));
#8412=CARTESIAN_POINT('Origin',(0.,-2.4,4.6));
#8413=CARTESIAN_POINT('',(2.2,-2.4,2.8));
#8414=CARTESIAN_POINT('',(0.,-2.4,2.8));
#8415=CARTESIAN_POINT('',(2.2,-2.4,6.5));
#8416=CARTESIAN_POINT('',(2.2,-2.4,2.7));
#8417=CARTESIAN_POINT('',(2.2,-2.4,6.5));
#8418=CARTESIAN_POINT('Origin',(0.,-2.4,4.6));
#8419=CARTESIAN_POINT('',(-1.15996323728161,-2.4,6.5));
#8420=CARTESIAN_POINT('',(2.2,-2.4,6.5));
#8421=CARTESIAN_POINT('',(-1.15996323728161,-2.4,2.8));
#8422=CARTESIAN_POINT('',(-1.15996323728161,-2.4,2.8));
#8423=CARTESIAN_POINT('',(0.,-2.4,2.8));
#8424=CARTESIAN_POINT('',(-0.505,-2.4,4.5));
#8425=CARTESIAN_POINT('Origin',(0.,-2.4,4.5));
#8426=CARTESIAN_POINT('Origin',(-2.2,-2.4,6.5));
#8427=CARTESIAN_POINT('',(2.2,-1.6,6.5));
#8428=CARTESIAN_POINT('',(2.2,-2.4,6.5));
#8429=CARTESIAN_POINT('',(2.2,-1.6,6.5));
#8430=CARTESIAN_POINT('Origin',(-2.2,-2.4,6.5));
#8431=CARTESIAN_POINT('',(-1.15996323728161,-1.6,6.5));
#8432=CARTESIAN_POINT('',(2.2,-1.6,6.5));
#8433=CARTESIAN_POINT('Origin',(-1.5,-2.,6.5));
#8434=CARTESIAN_POINT('Origin',(0.,-1.6,4.6));
#8435=CARTESIAN_POINT('',(2.2,-1.6,2.8));
#8436=CARTESIAN_POINT('',(2.2,-1.6,2.7));
#8437=CARTESIAN_POINT('',(0.,-1.6,2.8));
#8438=CARTESIAN_POINT('Origin',(0.,-1.6,4.6));
#8439=CARTESIAN_POINT('',(-1.15996323728161,-1.6,2.8));
#8440=CARTESIAN_POINT('',(0.,-1.6,2.8));
#8441=CARTESIAN_POINT('',(-1.15996323728161,-1.6,2.8));
#8442=CARTESIAN_POINT('',(-0.505,-1.6,4.5));
#8443=CARTESIAN_POINT('Origin',(0.,-1.6,4.5));
#8444=CARTESIAN_POINT('Origin',(1.5,-2.,1.9));
#8445=CARTESIAN_POINT('',(1.225,-2.,2.));
#8446=CARTESIAN_POINT('Origin',(1.5,-2.,2.));
#8447=CARTESIAN_POINT('',(1.225,-2.,2.8));
#8448=CARTESIAN_POINT('',(1.225,-2.,1.9));
#8449=CARTESIAN_POINT('Origin',(1.5,-2.,2.8));
#8450=CARTESIAN_POINT('Origin',(-1.5,-2.,2.8));
#8451=CARTESIAN_POINT('',(-1.84003676271839,-1.6,6.5));
#8452=CARTESIAN_POINT('',(-1.84003676271839,-1.6,2.8));
#8453=CARTESIAN_POINT('',(-1.84003676271839,-1.6,2.8));
#8454=CARTESIAN_POINT('',(-1.84003676271839,-2.4,6.5));
#8455=CARTESIAN_POINT('Origin',(-1.5,-2.,6.5));
#8456=CARTESIAN_POINT('',(-1.84003676271839,-2.4,2.8));
#8457=CARTESIAN_POINT('',(-1.84003676271839,-2.4,2.8));
#8458=CARTESIAN_POINT('Origin',(-1.5,-2.,2.8));
#8459=CARTESIAN_POINT('Origin',(-1.5,-2.,2.8));
#8460=CARTESIAN_POINT('Origin',(-1.5,-2.,2.8));
#8461=CARTESIAN_POINT('Origin',(0.,-1.6,4.6));
#8462=CARTESIAN_POINT('',(-2.2,-1.6,2.8));
#8463=CARTESIAN_POINT('',(0.,-1.6,2.8));
#8464=CARTESIAN_POINT('',(-2.2,-1.6,6.5));
#8465=CARTESIAN_POINT('',(-2.2,-1.6,6.5));
#8466=CARTESIAN_POINT('',(2.2,-1.6,6.5));
#8467=CARTESIAN_POINT('Origin',(-2.2,-2.4,6.5));
#8468=CARTESIAN_POINT('',(-2.2,-2.4,6.5));
#8469=CARTESIAN_POINT('',(-2.2,-2.4,6.5));
#8470=CARTESIAN_POINT('',(2.2,-2.4,6.5));
#8471=CARTESIAN_POINT('Origin',(0.,-2.4,4.6));
#8472=CARTESIAN_POINT('',(-2.2,-2.4,2.8));
#8473=CARTESIAN_POINT('',(-2.2,-2.4,6.5));
#8474=CARTESIAN_POINT('',(0.,-2.4,2.8));
#8475=CARTESIAN_POINT('Origin',(-1.5,-2.,1.9));
#8476=CARTESIAN_POINT('',(-1.775,-2.,2.));
#8477=CARTESIAN_POINT('Origin',(-1.5,-2.,2.));
#8478=CARTESIAN_POINT('',(-1.775,-2.,2.8));
#8479=CARTESIAN_POINT('',(-1.775,-2.,1.9));
#8480=CARTESIAN_POINT('Origin',(-1.5,-2.,2.8));
#8481=CARTESIAN_POINT('Origin',(0.,-2.5,4.5));
#8482=CARTESIAN_POINT('',(-0.505,-2.5,4.5));
#8483=CARTESIAN_POINT('Origin',(2.2,-2.4,6.5));
#8484=CARTESIAN_POINT('',(2.2,-2.2,2.8));
#8485=CARTESIAN_POINT('Origin',(-2.2,-2.4,2.7));
#8486=CARTESIAN_POINT('',(-2.2,-2.2,2.8));
#8487=CARTESIAN_POINT('Origin',(3.,-0.8,2.));
#8488=CARTESIAN_POINT('',(3.,-0.8,2.));
#8489=CARTESIAN_POINT('',(-3.,-0.8,2.));
#8490=CARTESIAN_POINT('',(3.,-0.8,2.));
#8491=CARTESIAN_POINT('',(-3.,-0.8,2.8));
#8492=CARTESIAN_POINT('',(-3.,-0.8,2.));
#8493=CARTESIAN_POINT('',(3.,-0.8,2.8));
#8494=CARTESIAN_POINT('',(3.,-0.8,2.8));
#8495=CARTESIAN_POINT('',(3.,-0.8,2.));
#8496=CARTESIAN_POINT('Origin',(3.,-3.2,2.));
#8497=CARTESIAN_POINT('',(3.,-3.2,2.));
#8498=CARTESIAN_POINT('',(3.,-3.2,2.));
#8499=CARTESIAN_POINT('',(3.,-3.2,2.8));
#8500=CARTESIAN_POINT('',(3.,-3.2,2.8));
#8501=CARTESIAN_POINT('',(3.,-3.2,2.));
#8502=CARTESIAN_POINT('Origin',(-3.,-3.2,2.));
#8503=CARTESIAN_POINT('',(-3.,-3.2,2.));
#8504=CARTESIAN_POINT('',(-3.,-3.2,2.));
#8505=CARTESIAN_POINT('',(-3.,-3.2,2.8));
#8506=CARTESIAN_POINT('',(-3.,-3.2,2.8));
#8507=CARTESIAN_POINT('',(-3.,-3.2,2.));
#8508=CARTESIAN_POINT('Origin',(-3.,-0.8,2.));
#8509=CARTESIAN_POINT('',(-3.,-0.8,2.));
#8510=CARTESIAN_POINT('',(-3.,-0.8,2.8));
#8511=CARTESIAN_POINT('Origin',(0.,-2.,2.8));
#8512=CARTESIAN_POINT('Origin',(0.,-2.,2.));
#9576=UNCERTAINTY_MEASURE_WITH_UNIT(LENGTH_MEASURE(0.001),#9623,
'DISTANCE_ACCURACY_VALUE',
'Maximum model space distance between geometric entities at asserted c
onnectivities');
#9592=UNCERTAINTY_MEASURE_WITH_UNIT(LENGTH_MEASURE(0.001),#9623,
'DISTANCE_ACCURACY_VALUE',
'Maximum model space distance between geometric entities at asserted c
onnectivities');
#9606=(
GEOMETRIC_REPRESENTATION_CONTEXT(3)
GLOBAL_UNCERTAINTY_ASSIGNED_CONTEXT((#9576))
GLOBAL_UNIT_ASSIGNED_CONTEXT((#9623,#9625,#9626))
REPRESENTATION_CONTEXT('','3D')
);
#9622=(
GEOMETRIC_REPRESENTATION_CONTEXT(3)
GLOBAL_UNCERTAINTY_ASSIGNED_CONTEXT((#9592))
GLOBAL_UNIT_ASSIGNED_CONTEXT((#9623,#9625,#9626))
REPRESENTATION_CONTEXT('','3D')
);
#9623=(
LENGTH_UNIT()
NAMED_UNIT(*)
SI_UNIT(.CENTI.,.METRE.)
);
#9625=(
NAMED_UNIT(*)
PLANE_ANGLE_UNIT()
SI_UNIT($,.RADIAN.)
);
#9626=(
NAMED_UNIT(*)
SI_UNIT($,.STERADIAN.)
SOLID_ANGLE_UNIT()
);
#9640=SHAPE_DEFINITION_REPRESENTATION(#9674,#9757);
#9674=PRODUCT_DEFINITION_SHAPE('',$,#9787);
#9757=SHAPE_REPRESENTATION('',(#5703),#9606);
#9773=PRODUCT_DEFINITION_CONTEXT('part definition',#9862,'design');
#9787=PRODUCT_DEFINITION('Sliding axle block','Sliding axle block',#9816,
#9773);
#9816=PRODUCT_DEFINITION_FORMATION('',$,#9877);
#9862=APPLICATION_CONTEXT(
'Core Data for Automotive Mechanical Design Process');
#9863=PRODUCT_CONTEXT('part definition',#9862,'mechanical');
#9877=PRODUCT('Sliding axle block','Sliding axle block',
'Sliding axle block',(#9863));
#9956=COLOUR_RGB('Grey',0.48,0.52,0.57);
#9957=FILL_AREA_STYLE_COLOUR('',#9956);
#9958=FILL_AREA_STYLE('',(#9957));
#9959=SURFACE_STYLE_FILL_AREA(#9958);
#9960=SURFACE_SIDE_STYLE('',(#9959));
#9961=SURFACE_STYLE_USAGE(.BOTH.,#9960);
#9962=PRESENTATION_STYLE_ASSIGNMENT((#9961));
ENDSEC;
END-ISO-10303-21;
